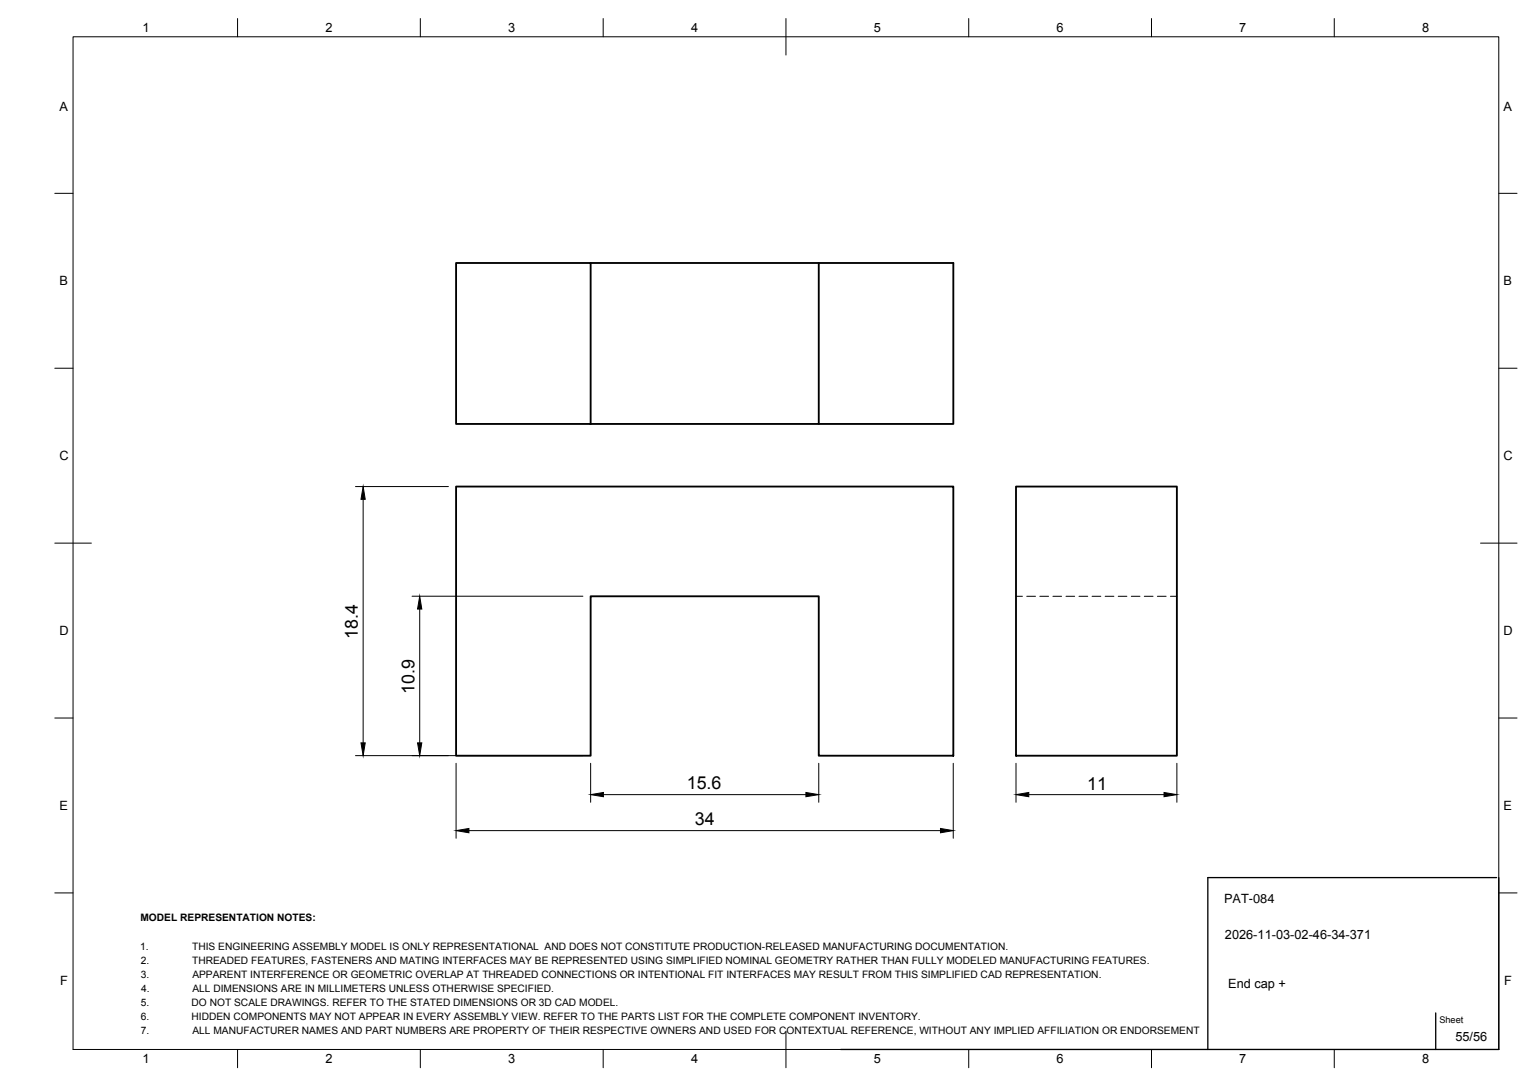
ISO-10303-21;
HEADER;
/* Generated by software containing ST-Developer
 * from STEP Tools, Inc. (www.steptools.com) 
 */

FILE_DESCRIPTION(
/* description */ ('Quick-return (Whitworth) mechanism'),
/* implementation_level */ '2;1');

FILE_NAME(
/* name */ 'End cap +.step',
/* time_stamp */ '2026-10-28T03:25:57-07:00',
/* author */ (''),
/* organization */ (''),
/* preprocessor_version */ 'ST-DEVELOPER v20.2',
/* originating_system */ 'Autodesk Translation Framework v15.17.0.0',
/* authorisation */ '');

FILE_SCHEMA (('AUTOMOTIVE_DESIGN { 1 0 10303 214 3 1 1 }'));
ENDSEC;

DATA;
#10=MECHANICAL_DESIGN_GEOMETRIC_PRESENTATION_REPRESENTATION('',(#538),#14878);
#442=SHAPE_REPRESENTATION_RELATIONSHIP('SRR','None',#15117,#486);
#486=ADVANCED_BREP_SHAPE_REPRESENTATION('',(#589),#14874);
#538=STYLED_ITEM('',(#15399),#589);
#589=MANIFOLD_SOLID_BREP('Body1',#7893);
#1005=PLANE('',#9258);
#1006=PLANE('',#9259);
#1007=PLANE('',#9260);
#1008=PLANE('',#9261);
#1009=PLANE('',#9262);
#1010=PLANE('',#9263);
#1011=PLANE('',#9264);
#1012=PLANE('',#9265);
#1013=PLANE('',#9266);
#1014=PLANE('',#9267);
#1461=FACE_OUTER_BOUND('',#2116,.T.);
#1462=FACE_OUTER_BOUND('',#2117,.T.);
#1463=FACE_OUTER_BOUND('',#2118,.T.);
#1464=FACE_OUTER_BOUND('',#2119,.T.);
#1465=FACE_OUTER_BOUND('',#2120,.T.);
#1466=FACE_OUTER_BOUND('',#2121,.T.);
#1467=FACE_OUTER_BOUND('',#2122,.T.);
#1468=FACE_OUTER_BOUND('',#2123,.T.);
#1469=FACE_OUTER_BOUND('',#2124,.T.);
#1470=FACE_OUTER_BOUND('',#2125,.T.);
#2116=EDGE_LOOP('',(#6994,#6995,#6996,#6997));
#2117=EDGE_LOOP('',(#6998,#6999,#7000,#7001));
#2118=EDGE_LOOP('',(#7002,#7003,#7004,#7005));
#2119=EDGE_LOOP('',(#7006,#7007,#7008,#7009));
#2120=EDGE_LOOP('',(#7010,#7011,#7012,#7013));
#2121=EDGE_LOOP('',(#7014,#7015,#7016,#7017));
#2122=EDGE_LOOP('',(#7018,#7019,#7020,#7021));
#2123=EDGE_LOOP('',(#7022,#7023,#7024,#7025));
#2124=EDGE_LOOP('',(#7026,#7027,#7028,#7029,#7030,#7031,#7032,#7033));
#2125=EDGE_LOOP('',(#7034,#7035,#7036,#7037,#7038,#7039,#7040,#7041));
#2599=LINE('',#14471,#3122);
#2600=LINE('',#14473,#3123);
#2601=LINE('',#14475,#3124);
#2602=LINE('',#14476,#3125);
#2603=LINE('',#14479,#3126);
#2604=LINE('',#14481,#3127);
#2605=LINE('',#14482,#3128);
#2606=LINE('',#14485,#3129);
#2607=LINE('',#14487,#3130);
#2608=LINE('',#14488,#3131);
#2609=LINE('',#14491,#3132);
#2610=LINE('',#14493,#3133);
#2611=LINE('',#14494,#3134);
#2612=LINE('',#14497,#3135);
#2613=LINE('',#14499,#3136);
#2614=LINE('',#14500,#3137);
#2615=LINE('',#14503,#3138);
#2616=LINE('',#14505,#3139);
#2617=LINE('',#14506,#3140);
#2618=LINE('',#14509,#3141);
#2619=LINE('',#14511,#3142);
#2620=LINE('',#14512,#3143);
#2621=LINE('',#14514,#3144);
#2622=LINE('',#14515,#3145);
#3122=VECTOR('',#11576,1.);
#3123=VECTOR('',#11577,1.);
#3124=VECTOR('',#11578,1.);
#3125=VECTOR('',#11579,1.);
#3126=VECTOR('',#11582,1.);
#3127=VECTOR('',#11583,1.);
#3128=VECTOR('',#11584,1.);
#3129=VECTOR('',#11587,1.);
#3130=VECTOR('',#11588,1.);
#3131=VECTOR('',#11589,1.);
#3132=VECTOR('',#11592,1.);
#3133=VECTOR('',#11593,1.);
#3134=VECTOR('',#11594,1.);
#3135=VECTOR('',#11597,1.);
#3136=VECTOR('',#11598,1.);
#3137=VECTOR('',#11599,1.);
#3138=VECTOR('',#11602,1.);
#3139=VECTOR('',#11603,1.);
#3140=VECTOR('',#11604,1.);
#3141=VECTOR('',#11607,1.);
#3142=VECTOR('',#11608,1.);
#3143=VECTOR('',#11609,1.);
#3144=VECTOR('',#11612,1.);
#3145=VECTOR('',#11613,1.);
#4218=VERTEX_POINT('',#14469);
#4219=VERTEX_POINT('',#14470);
#4220=VERTEX_POINT('',#14472);
#4221=VERTEX_POINT('',#14474);
#4222=VERTEX_POINT('',#14478);
#4223=VERTEX_POINT('',#14480);
#4224=VERTEX_POINT('',#14484);
#4225=VERTEX_POINT('',#14486);
#4226=VERTEX_POINT('',#14490);
#4227=VERTEX_POINT('',#14492);
#4228=VERTEX_POINT('',#14496);
#4229=VERTEX_POINT('',#14498);
#4230=VERTEX_POINT('',#14502);
#4231=VERTEX_POINT('',#14504);
#4232=VERTEX_POINT('',#14508);
#4233=VERTEX_POINT('',#14510);
#5154=EDGE_CURVE('',#4218,#4219,#2599,.T.);
#5155=EDGE_CURVE('',#4219,#4220,#2600,.T.);
#5156=EDGE_CURVE('',#4221,#4220,#2601,.T.);
#5157=EDGE_CURVE('',#4218,#4221,#2602,.T.);
#5158=EDGE_CURVE('',#4222,#4218,#2603,.T.);
#5159=EDGE_CURVE('',#4223,#4221,#2604,.T.);
#5160=EDGE_CURVE('',#4222,#4223,#2605,.T.);
#5161=EDGE_CURVE('',#4224,#4222,#2606,.T.);
#5162=EDGE_CURVE('',#4225,#4223,#2607,.T.);
#5163=EDGE_CURVE('',#4224,#4225,#2608,.T.);
#5164=EDGE_CURVE('',#4226,#4224,#2609,.T.);
#5165=EDGE_CURVE('',#4227,#4225,#2610,.T.);
#5166=EDGE_CURVE('',#4226,#4227,#2611,.T.);
#5167=EDGE_CURVE('',#4228,#4226,#2612,.T.);
#5168=EDGE_CURVE('',#4229,#4227,#2613,.T.);
#5169=EDGE_CURVE('',#4228,#4229,#2614,.T.);
#5170=EDGE_CURVE('',#4230,#4228,#2615,.T.);
#5171=EDGE_CURVE('',#4231,#4229,#2616,.T.);
#5172=EDGE_CURVE('',#4230,#4231,#2617,.T.);
#5173=EDGE_CURVE('',#4232,#4230,#2618,.T.);
#5174=EDGE_CURVE('',#4233,#4231,#2619,.T.);
#5175=EDGE_CURVE('',#4232,#4233,#2620,.T.);
#5176=EDGE_CURVE('',#4219,#4232,#2621,.T.);
#5177=EDGE_CURVE('',#4220,#4233,#2622,.T.);
#6994=ORIENTED_EDGE('',*,*,#5154,.T.);
#6995=ORIENTED_EDGE('',*,*,#5155,.T.);
#6996=ORIENTED_EDGE('',*,*,#5156,.F.);
#6997=ORIENTED_EDGE('',*,*,#5157,.F.);
#6998=ORIENTED_EDGE('',*,*,#5158,.T.);
#6999=ORIENTED_EDGE('',*,*,#5157,.T.);
#7000=ORIENTED_EDGE('',*,*,#5159,.F.);
#7001=ORIENTED_EDGE('',*,*,#5160,.F.);
#7002=ORIENTED_EDGE('',*,*,#5161,.T.);
#7003=ORIENTED_EDGE('',*,*,#5160,.T.);
#7004=ORIENTED_EDGE('',*,*,#5162,.F.);
#7005=ORIENTED_EDGE('',*,*,#5163,.F.);
#7006=ORIENTED_EDGE('',*,*,#5164,.T.);
#7007=ORIENTED_EDGE('',*,*,#5163,.T.);
#7008=ORIENTED_EDGE('',*,*,#5165,.F.);
#7009=ORIENTED_EDGE('',*,*,#5166,.F.);
#7010=ORIENTED_EDGE('',*,*,#5167,.T.);
#7011=ORIENTED_EDGE('',*,*,#5166,.T.);
#7012=ORIENTED_EDGE('',*,*,#5168,.F.);
#7013=ORIENTED_EDGE('',*,*,#5169,.F.);
#7014=ORIENTED_EDGE('',*,*,#5170,.T.);
#7015=ORIENTED_EDGE('',*,*,#5169,.T.);
#7016=ORIENTED_EDGE('',*,*,#5171,.F.);
#7017=ORIENTED_EDGE('',*,*,#5172,.F.);
#7018=ORIENTED_EDGE('',*,*,#5173,.T.);
#7019=ORIENTED_EDGE('',*,*,#5172,.T.);
#7020=ORIENTED_EDGE('',*,*,#5174,.F.);
#7021=ORIENTED_EDGE('',*,*,#5175,.F.);
#7022=ORIENTED_EDGE('',*,*,#5176,.T.);
#7023=ORIENTED_EDGE('',*,*,#5175,.T.);
#7024=ORIENTED_EDGE('',*,*,#5177,.F.);
#7025=ORIENTED_EDGE('',*,*,#5155,.F.);
#7026=ORIENTED_EDGE('',*,*,#5177,.T.);
#7027=ORIENTED_EDGE('',*,*,#5174,.T.);
#7028=ORIENTED_EDGE('',*,*,#5171,.T.);
#7029=ORIENTED_EDGE('',*,*,#5168,.T.);
#7030=ORIENTED_EDGE('',*,*,#5165,.T.);
#7031=ORIENTED_EDGE('',*,*,#5162,.T.);
#7032=ORIENTED_EDGE('',*,*,#5159,.T.);
#7033=ORIENTED_EDGE('',*,*,#5156,.T.);
#7034=ORIENTED_EDGE('',*,*,#5176,.F.);
#7035=ORIENTED_EDGE('',*,*,#5154,.F.);
#7036=ORIENTED_EDGE('',*,*,#5158,.F.);
#7037=ORIENTED_EDGE('',*,*,#5161,.F.);
#7038=ORIENTED_EDGE('',*,*,#5164,.F.);
#7039=ORIENTED_EDGE('',*,*,#5167,.F.);
#7040=ORIENTED_EDGE('',*,*,#5170,.F.);
#7041=ORIENTED_EDGE('',*,*,#5173,.F.);
#7792=ADVANCED_FACE('',(#1461),#1005,.T.);
#7793=ADVANCED_FACE('',(#1462),#1006,.T.);
#7794=ADVANCED_FACE('',(#1463),#1007,.T.);
#7795=ADVANCED_FACE('',(#1464),#1008,.T.);
#7796=ADVANCED_FACE('',(#1465),#1009,.T.);
#7797=ADVANCED_FACE('',(#1466),#1010,.T.);
#7798=ADVANCED_FACE('',(#1467),#1011,.T.);
#7799=ADVANCED_FACE('',(#1468),#1012,.T.);
#7800=ADVANCED_FACE('',(#1469),#1013,.T.);
#7801=ADVANCED_FACE('',(#1470),#1014,.F.);
#7893=CLOSED_SHELL('',(#7792,#7793,#7794,#7795,#7796,#7797,#7798,#7799,
#7800,#7801));
#9257=AXIS2_PLACEMENT_3D('',#14467,#11572,#11573);
#9258=AXIS2_PLACEMENT_3D('',#14468,#11574,#11575);
#9259=AXIS2_PLACEMENT_3D('',#14477,#11580,#11581);
#9260=AXIS2_PLACEMENT_3D('',#14483,#11585,#11586);
#9261=AXIS2_PLACEMENT_3D('',#14489,#11590,#11591);
#9262=AXIS2_PLACEMENT_3D('',#14495,#11595,#11596);
#9263=AXIS2_PLACEMENT_3D('',#14501,#11600,#11601);
#9264=AXIS2_PLACEMENT_3D('',#14507,#11605,#11606);
#9265=AXIS2_PLACEMENT_3D('',#14513,#11610,#11611);
#9266=AXIS2_PLACEMENT_3D('',#14516,#11614,#11615);
#9267=AXIS2_PLACEMENT_3D('',#14517,#11616,#11617);
#11572=DIRECTION('axis',(0.,0.,1.));
#11573=DIRECTION('refdir',(1.,0.,0.));
#11574=DIRECTION('center_axis',(0.,0.,1.));
#11575=DIRECTION('ref_axis',(0.,-1.,0.));
#11576=DIRECTION('',(0.,-1.,0.));
#11577=DIRECTION('',(1.,0.,0.));
#11578=DIRECTION('',(0.,-1.,0.));
#11579=DIRECTION('',(1.,0.,0.));
#11580=DIRECTION('center_axis',(0.,1.,0.));
#11581=DIRECTION('ref_axis',(0.,0.,1.));
#11582=DIRECTION('',(0.,0.,1.));
#11583=DIRECTION('',(0.,0.,1.));
#11584=DIRECTION('',(1.,0.,0.));
#11585=DIRECTION('center_axis',(0.,0.,-1.));
#11586=DIRECTION('ref_axis',(0.,1.,0.));
#11587=DIRECTION('',(0.,1.,0.));
#11588=DIRECTION('',(0.,1.,0.));
#11589=DIRECTION('',(1.,0.,0.));
#11590=DIRECTION('center_axis',(0.,-1.,0.));
#11591=DIRECTION('ref_axis',(0.,0.,-1.));
#11592=DIRECTION('',(0.,0.,-1.));
#11593=DIRECTION('',(0.,0.,-1.));
#11594=DIRECTION('',(1.,0.,0.));
#11595=DIRECTION('center_axis',(0.,0.,-1.));
#11596=DIRECTION('ref_axis',(0.,1.,0.));
#11597=DIRECTION('',(0.,1.,0.));
#11598=DIRECTION('',(0.,1.,0.));
#11599=DIRECTION('',(1.,0.,0.));
#11600=DIRECTION('center_axis',(0.,1.,0.));
#11601=DIRECTION('ref_axis',(0.,0.,1.));
#11602=DIRECTION('',(0.,0.,1.));
#11603=DIRECTION('',(0.,0.,1.));
#11604=DIRECTION('',(1.,0.,0.));
#11605=DIRECTION('center_axis',(0.,0.,-1.));
#11606=DIRECTION('ref_axis',(0.,1.,0.));
#11607=DIRECTION('',(0.,1.,0.));
#11608=DIRECTION('',(0.,1.,0.));
#11609=DIRECTION('',(1.,0.,0.));
#11610=DIRECTION('center_axis',(0.,-1.,0.));
#11611=DIRECTION('ref_axis',(0.,0.,-1.));
#11612=DIRECTION('',(0.,0.,-1.));
#11613=DIRECTION('',(0.,0.,-1.));
#11614=DIRECTION('center_axis',(1.,0.,0.));
#11615=DIRECTION('ref_axis',(0.,0.,-1.));
#11616=DIRECTION('center_axis',(1.,0.,0.));
#11617=DIRECTION('ref_axis',(0.,0.,-1.));
#14467=CARTESIAN_POINT('',(0.,0.,0.));
#14468=CARTESIAN_POINT('Origin',(1.97,1.7,2.3));
#14469=CARTESIAN_POINT('',(1.97,1.7,2.3));
#14470=CARTESIAN_POINT('',(1.97,-1.7,2.3));
#14471=CARTESIAN_POINT('',(1.97,1.7,2.3));
#14472=CARTESIAN_POINT('',(3.07,-1.7,2.3));
#14473=CARTESIAN_POINT('',(1.97,-1.7,2.3));
#14474=CARTESIAN_POINT('',(3.07,1.7,2.3));
#14475=CARTESIAN_POINT('',(3.07,1.7,2.3));
#14476=CARTESIAN_POINT('',(1.97,1.7,2.3));
#14477=CARTESIAN_POINT('Origin',(1.97,1.7,0.46));
#14478=CARTESIAN_POINT('',(1.97,1.7,0.46));
#14479=CARTESIAN_POINT('',(1.97,1.7,0.46));
#14480=CARTESIAN_POINT('',(3.07,1.7,0.46));
#14481=CARTESIAN_POINT('',(3.07,1.7,0.46));
#14482=CARTESIAN_POINT('',(1.97,1.7,0.46));
#14483=CARTESIAN_POINT('Origin',(1.97,0.78,0.46));
#14484=CARTESIAN_POINT('',(1.97,0.78,0.46));
#14485=CARTESIAN_POINT('',(1.97,0.78,0.46));
#14486=CARTESIAN_POINT('',(3.07,0.78,0.46));
#14487=CARTESIAN_POINT('',(3.07,0.78,0.46));
#14488=CARTESIAN_POINT('',(1.97,0.78,0.46));
#14489=CARTESIAN_POINT('Origin',(1.97,0.78,1.55));
#14490=CARTESIAN_POINT('',(1.97,0.78,1.55));
#14491=CARTESIAN_POINT('',(1.97,0.78,1.55));
#14492=CARTESIAN_POINT('',(3.07,0.78,1.55));
#14493=CARTESIAN_POINT('',(3.07,0.78,1.55));
#14494=CARTESIAN_POINT('',(1.97,0.78,1.55));
#14495=CARTESIAN_POINT('Origin',(1.97,-0.78,1.55));
#14496=CARTESIAN_POINT('',(1.97,-0.78,1.55));
#14497=CARTESIAN_POINT('',(1.97,-0.78,1.55));
#14498=CARTESIAN_POINT('',(3.07,-0.78,1.55));
#14499=CARTESIAN_POINT('',(3.07,-0.78,1.55));
#14500=CARTESIAN_POINT('',(1.97,-0.78,1.55));
#14501=CARTESIAN_POINT('Origin',(1.97,-0.78,0.46));
#14502=CARTESIAN_POINT('',(1.97,-0.78,0.46));
#14503=CARTESIAN_POINT('',(1.97,-0.78,0.46));
#14504=CARTESIAN_POINT('',(3.07,-0.78,0.46));
#14505=CARTESIAN_POINT('',(3.07,-0.78,0.46));
#14506=CARTESIAN_POINT('',(1.97,-0.78,0.46));
#14507=CARTESIAN_POINT('Origin',(1.97,-1.7,0.46));
#14508=CARTESIAN_POINT('',(1.97,-1.7,0.46));
#14509=CARTESIAN_POINT('',(1.97,-1.7,0.46));
#14510=CARTESIAN_POINT('',(3.07,-1.7,0.46));
#14511=CARTESIAN_POINT('',(3.07,-1.7,0.46));
#14512=CARTESIAN_POINT('',(1.97,-1.7,0.46));
#14513=CARTESIAN_POINT('Origin',(1.97,-1.7,2.3));
#14514=CARTESIAN_POINT('',(1.97,-1.7,2.3));
#14515=CARTESIAN_POINT('',(3.07,-1.7,2.3));
#14516=CARTESIAN_POINT('Origin',(3.07,0.,1.38));
#14517=CARTESIAN_POINT('Origin',(1.97,0.,1.38));
#14820=UNCERTAINTY_MEASURE_WITH_UNIT(LENGTH_MEASURE(0.001),#14879,
'DISTANCE_ACCURACY_VALUE',
'Maximum model space distance between geometric entities at asserted c
onnectivities');
#14824=UNCERTAINTY_MEASURE_WITH_UNIT(LENGTH_MEASURE(0.001),#14879,
'DISTANCE_ACCURACY_VALUE',
'Maximum model space distance between geometric entities at asserted c
onnectivities');
#14874=(
GEOMETRIC_REPRESENTATION_CONTEXT(3)
GLOBAL_UNCERTAINTY_ASSIGNED_CONTEXT((#14820))
GLOBAL_UNIT_ASSIGNED_CONTEXT((#14879,#14881,#14882))
REPRESENTATION_CONTEXT('','3D')
);
#14878=(
GEOMETRIC_REPRESENTATION_CONTEXT(3)
GLOBAL_UNCERTAINTY_ASSIGNED_CONTEXT((#14824))
GLOBAL_UNIT_ASSIGNED_CONTEXT((#14879,#14881,#14882))
REPRESENTATION_CONTEXT('','3D')
);
#14879=(
LENGTH_UNIT()
NAMED_UNIT(*)
SI_UNIT(.CENTI.,.METRE.)
);
#14881=(
NAMED_UNIT(*)
PLANE_ANGLE_UNIT()
SI_UNIT($,.RADIAN.)
);
#14882=(
NAMED_UNIT(*)
SI_UNIT($,.STERADIAN.)
SOLID_ANGLE_UNIT()
);
#14932=SHAPE_DEFINITION_REPRESENTATION(#14994,#15117);
#14994=PRODUCT_DEFINITION_SHAPE('',$,#15171);
#15117=SHAPE_REPRESENTATION('',(#9257),#14874);
#15121=PRODUCT_DEFINITION_CONTEXT('part definition',#15282,'design');
#15171=PRODUCT_DEFINITION('End cap +','End cap +',#15224,#15121);
#15224=PRODUCT_DEFINITION_FORMATION('',$,#15333);
#15282=APPLICATION_CONTEXT(
'Core Data for Automotive Mechanical Design Process');
#15283=PRODUCT_CONTEXT('part definition',#15282,'mechanical');
#15333=PRODUCT('End cap +','End cap +','End cap +',(#15283));
#15393=COLOUR_RGB('Sky Blue',0.24,0.69,0.87);
#15394=FILL_AREA_STYLE_COLOUR('',#15393);
#15395=FILL_AREA_STYLE('',(#15394));
#15396=SURFACE_STYLE_FILL_AREA(#15395);
#15397=SURFACE_SIDE_STYLE('',(#15396));
#15398=SURFACE_STYLE_USAGE(.BOTH.,#15397);
#15399=PRESENTATION_STYLE_ASSIGNMENT((#15398));
ENDSEC;
END-ISO-10303-21;
